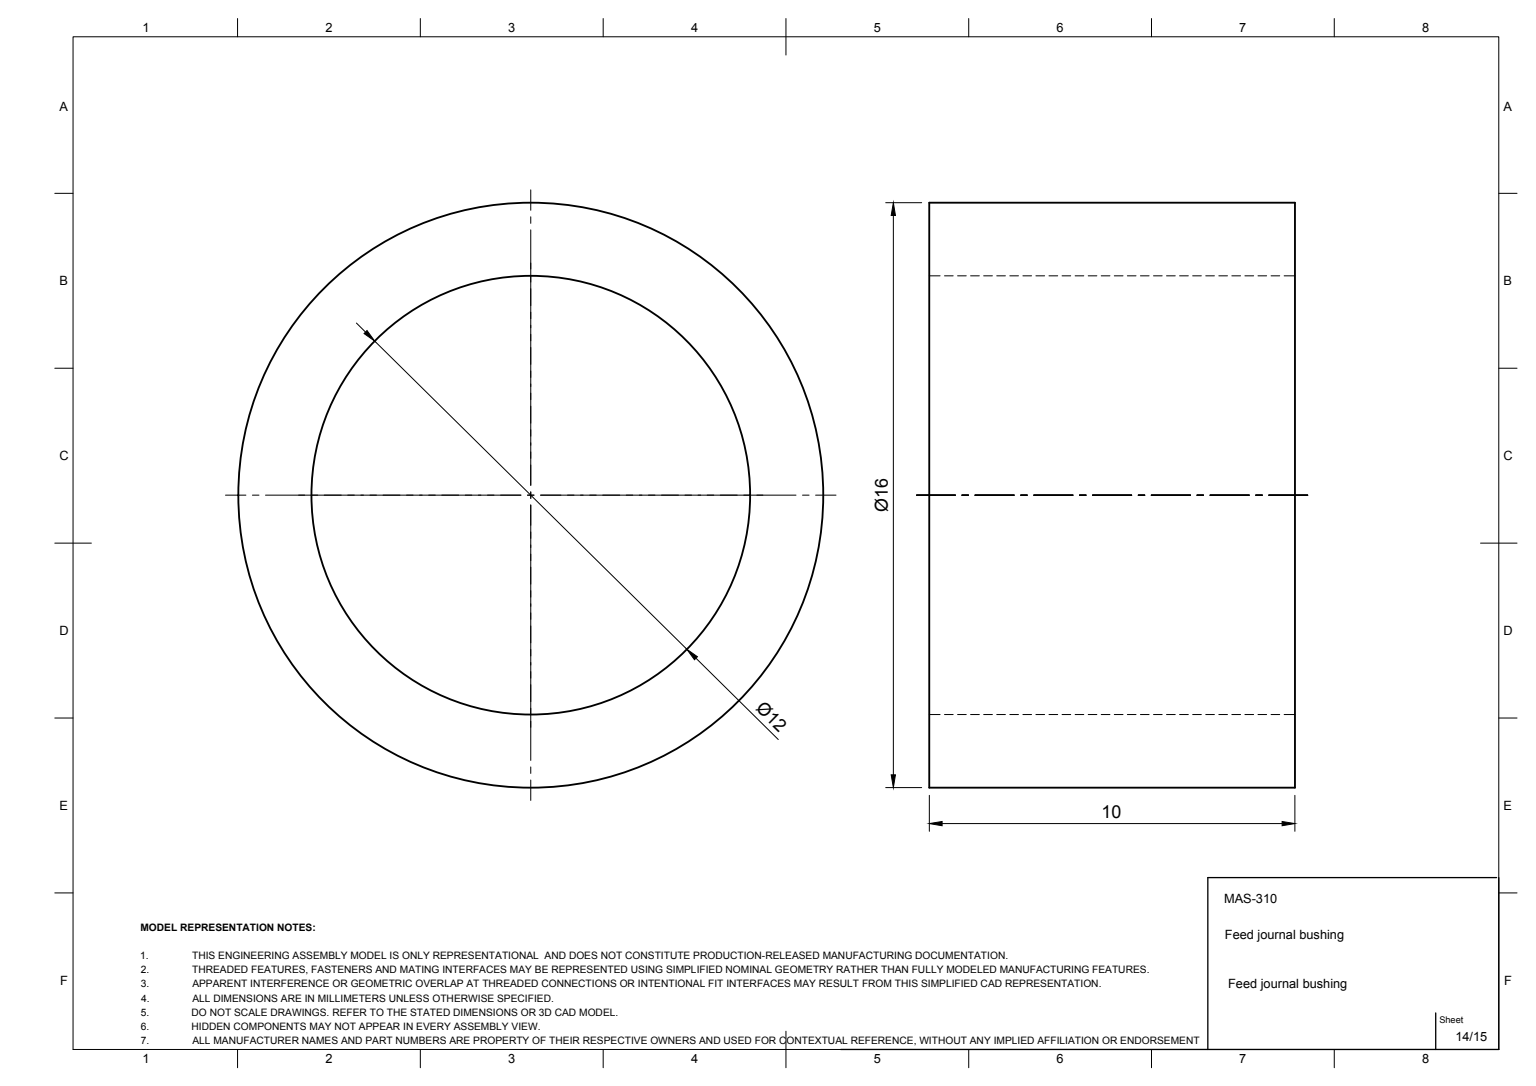
ISO-10303-21;
HEADER;
/* Generated by software containing ST-Developer
 * from STEP Tools, Inc. (www.steptools.com) 
 */

FILE_DESCRIPTION(
/* description */ ('Independent30mm screw-fed quill/spindle unit with16mm straight tool s
ocket, radial set screw, native reusable open ball bearings, retained 
inner/outer race stacks, keyed quill guide and M12x1.75 fine feed. Ext
ernal moving drive and tool not included. Ideal cage orbital links; in
dividual ball spin, force and preload not simulated. No drilling capac
ity, runout, speed, torque, load, life or machine safety rating.'),
/* implementation_level */ '2;1');

FILE_NAME(
/* name */ 'Feed journal bushing.step',
/* time_stamp */ '2026-11-08T18:59:42-08:00',
/* author */ (''),
/* organization */ (''),
/* preprocessor_version */ 'ST-DEVELOPER v20.2',
/* originating_system */ 'Autodesk Translation Framework v15.17.0.0',
/* authorisation */ '');

FILE_SCHEMA (('AUTOMOTIVE_DESIGN { 1 0 10303 214 3 1 1 }'));
ENDSEC;

DATA;
#10=MECHANICAL_DESIGN_GEOMETRIC_PRESENTATION_REPRESENTATION('',(#1600),#63898);
#1564=SHAPE_REPRESENTATION_RELATIONSHIP('SRR','None',#64003,#1582);
#1582=ADVANCED_BREP_SHAPE_REPRESENTATION('',(#1618),#63888);
#1600=STYLED_ITEM('',(#64097),#1618);
#1618=MANIFOLD_SOLID_BREP('Body1',#15486);
#1689=FACE_BOUND('',#4233,.T.);
#1690=FACE_BOUND('',#4235,.T.);
#2283=CYLINDRICAL_SURFACE('',#16512,6.);
#2284=CYLINDRICAL_SURFACE('',#16515,8.);
#2538=CIRCLE('',#16513,6.);
#2539=CIRCLE('',#16514,6.);
#2540=CIRCLE('',#16516,8.);
#2541=CIRCLE('',#16517,8.);
#3331=FACE_OUTER_BOUND('',#4230,.T.);
#3332=FACE_OUTER_BOUND('',#4231,.T.);
#3333=FACE_OUTER_BOUND('',#4232,.T.);
#3334=FACE_OUTER_BOUND('',#4234,.T.);
#4230=EDGE_LOOP('',(#13618,#13619,#13620,#13621));
#4231=EDGE_LOOP('',(#13622,#13623,#13624,#13625));
#4232=EDGE_LOOP('',(#13626));
#4233=EDGE_LOOP('',(#13627));
#4234=EDGE_LOOP('',(#13628));
#4235=EDGE_LOOP('',(#13629));
#5050=LINE('',#57553,#5813);
#5051=LINE('',#57559,#5814);
#5813=VECTOR('',#19124,6.);
#5814=VECTOR('',#19131,8.);
#7206=VERTEX_POINT('',#57550);
#7207=VERTEX_POINT('',#57552);
#7208=VERTEX_POINT('',#57556);
#7209=VERTEX_POINT('',#57558);
#9398=EDGE_CURVE('',#7206,#7206,#2538,.T.);
#9399=EDGE_CURVE('',#7206,#7207,#5050,.T.);
#9400=EDGE_CURVE('',#7207,#7207,#2539,.T.);
#9401=EDGE_CURVE('',#7208,#7208,#2540,.T.);
#9402=EDGE_CURVE('',#7208,#7209,#5051,.T.);
#9403=EDGE_CURVE('',#7209,#7209,#2541,.T.);
#13618=ORIENTED_EDGE('',*,*,#9398,.F.);
#13619=ORIENTED_EDGE('',*,*,#9399,.T.);
#13620=ORIENTED_EDGE('',*,*,#9400,.T.);
#13621=ORIENTED_EDGE('',*,*,#9399,.F.);
#13622=ORIENTED_EDGE('',*,*,#9401,.F.);
#13623=ORIENTED_EDGE('',*,*,#9402,.T.);
#13624=ORIENTED_EDGE('',*,*,#9403,.T.);
#13625=ORIENTED_EDGE('',*,*,#9402,.F.);
#13626=ORIENTED_EDGE('',*,*,#9401,.T.);
#13627=ORIENTED_EDGE('',*,*,#9398,.T.);
#13628=ORIENTED_EDGE('',*,*,#9403,.F.);
#13629=ORIENTED_EDGE('',*,*,#9400,.F.);
#14590=PLANE('',#16518);
#14591=PLANE('',#16519);
#15311=ADVANCED_FACE('',(#3331),#2283,.F.);
#15312=ADVANCED_FACE('',(#3332),#2284,.T.);
#15313=ADVANCED_FACE('',(#3333,#1689),#14590,.T.);
#15314=ADVANCED_FACE('',(#3334,#1690),#14591,.F.);
#15486=CLOSED_SHELL('',(#15311,#15312,#15313,#15314));
#16511=AXIS2_PLACEMENT_3D('',#57548,#19118,#19119);
#16512=AXIS2_PLACEMENT_3D('',#57549,#19120,#19121);
#16513=AXIS2_PLACEMENT_3D('',#57551,#19122,#19123);
#16514=AXIS2_PLACEMENT_3D('',#57554,#19125,#19126);
#16515=AXIS2_PLACEMENT_3D('',#57555,#19127,#19128);
#16516=AXIS2_PLACEMENT_3D('',#57557,#19129,#19130);
#16517=AXIS2_PLACEMENT_3D('',#57560,#19132,#19133);
#16518=AXIS2_PLACEMENT_3D('',#57561,#19134,#19135);
#16519=AXIS2_PLACEMENT_3D('',#57562,#19136,#19137);
#19118=DIRECTION('axis',(0.,0.,1.));
#19119=DIRECTION('refdir',(1.,0.,0.));
#19120=DIRECTION('center_axis',(0.,0.,1.));
#19121=DIRECTION('ref_axis',(1.,0.,0.));
#19122=DIRECTION('center_axis',(0.,0.,-1.));
#19123=DIRECTION('ref_axis',(1.,0.,0.));
#19124=DIRECTION('',(0.,0.,-1.));
#19125=DIRECTION('center_axis',(0.,0.,-1.));
#19126=DIRECTION('ref_axis',(1.,0.,0.));
#19127=DIRECTION('center_axis',(0.,0.,1.));
#19128=DIRECTION('ref_axis',(1.,0.,0.));
#19129=DIRECTION('center_axis',(0.,0.,1.));
#19130=DIRECTION('ref_axis',(1.,0.,0.));
#19131=DIRECTION('',(0.,0.,-1.));
#19132=DIRECTION('center_axis',(0.,0.,1.));
#19133=DIRECTION('ref_axis',(1.,0.,0.));
#19134=DIRECTION('center_axis',(0.,0.,1.));
#19135=DIRECTION('ref_axis',(1.,0.,0.));
#19136=DIRECTION('center_axis',(0.,0.,1.));
#19137=DIRECTION('ref_axis',(1.,0.,0.));
#57548=CARTESIAN_POINT('',(0.,0.,0.));
#57549=CARTESIAN_POINT('Origin',(0.,0.,0.));
#57550=CARTESIAN_POINT('',(-6.,-7.34788079488412E-16,10.));
#57551=CARTESIAN_POINT('Origin',(0.,0.,10.));
#57552=CARTESIAN_POINT('',(-6.,-7.34788079488412E-16,0.));
#57553=CARTESIAN_POINT('',(-6.,-7.34788079488412E-16,0.));
#57554=CARTESIAN_POINT('Origin',(0.,0.,0.));
#57555=CARTESIAN_POINT('Origin',(0.,0.,0.));
#57556=CARTESIAN_POINT('',(-8.,-9.79717439317883E-16,10.));
#57557=CARTESIAN_POINT('Origin',(0.,0.,10.));
#57558=CARTESIAN_POINT('',(-8.,-9.79717439317883E-16,0.));
#57559=CARTESIAN_POINT('',(-8.,-9.79717439317883E-16,0.));
#57560=CARTESIAN_POINT('Origin',(0.,0.,0.));
#57561=CARTESIAN_POINT('Origin',(0.,0.,10.));
#57562=CARTESIAN_POINT('Origin',(0.,0.,0.));
#63868=UNCERTAINTY_MEASURE_WITH_UNIT(LENGTH_MEASURE(0.01),#63899,
'DISTANCE_ACCURACY_VALUE',
'Maximum model space distance between geometric entities at asserted c
onnectivities');
#63878=UNCERTAINTY_MEASURE_WITH_UNIT(LENGTH_MEASURE(0.01),#63899,
'DISTANCE_ACCURACY_VALUE',
'Maximum model space distance between geometric entities at asserted c
onnectivities');
#63888=(
GEOMETRIC_REPRESENTATION_CONTEXT(3)
GLOBAL_UNCERTAINTY_ASSIGNED_CONTEXT((#63868))
GLOBAL_UNIT_ASSIGNED_CONTEXT((#63899,#63901,#63902))
REPRESENTATION_CONTEXT('','3D')
);
#63898=(
GEOMETRIC_REPRESENTATION_CONTEXT(3)
GLOBAL_UNCERTAINTY_ASSIGNED_CONTEXT((#63878))
GLOBAL_UNIT_ASSIGNED_CONTEXT((#63899,#63901,#63902))
REPRESENTATION_CONTEXT('','3D')
);
#63899=(
LENGTH_UNIT()
NAMED_UNIT(*)
SI_UNIT(.MILLI.,.METRE.)
);
#63901=(
NAMED_UNIT(*)
PLANE_ANGLE_UNIT()
SI_UNIT($,.RADIAN.)
);
#63902=(
NAMED_UNIT(*)
SI_UNIT($,.STERADIAN.)
SOLID_ANGLE_UNIT()
);
#63912=SHAPE_DEFINITION_REPRESENTATION(#63931,#64003);
#63931=PRODUCT_DEFINITION_SHAPE('',$,#64023);
#64003=SHAPE_REPRESENTATION('',(#16511),#63888);
#64013=PRODUCT_DEFINITION_CONTEXT('part definition',#64072,'design');
#64023=PRODUCT_DEFINITION('Feed journal bushing','Feed journal bushing',
#64042,#64013);
#64042=PRODUCT_DEFINITION_FORMATION('',$,#64083);
#64072=APPLICATION_CONTEXT(
'Core Data for Automotive Mechanical Design Process');
#64073=PRODUCT_CONTEXT('part definition',#64072,'mechanical');
#64083=PRODUCT('Feed journal bushing','Feed journal bushing',$,(#64073));
#64097=PRESENTATION_STYLE_ASSIGNMENT((#64110));
#64110=SURFACE_STYLE_USAGE(.BOTH.,#64123);
#64123=SURFACE_SIDE_STYLE('',(#64136));
#64136=SURFACE_STYLE_FILL_AREA(#64149);
#64149=FILL_AREA_STYLE('Light gray',(#64162));
#64162=FILL_AREA_STYLE_COLOUR('Light gray',#64175);
#64175=COLOUR_RGB('Light gray',0.725490196078431,0.752941176470588,0.792156862745098);
ENDSEC;
END-ISO-10303-21;
